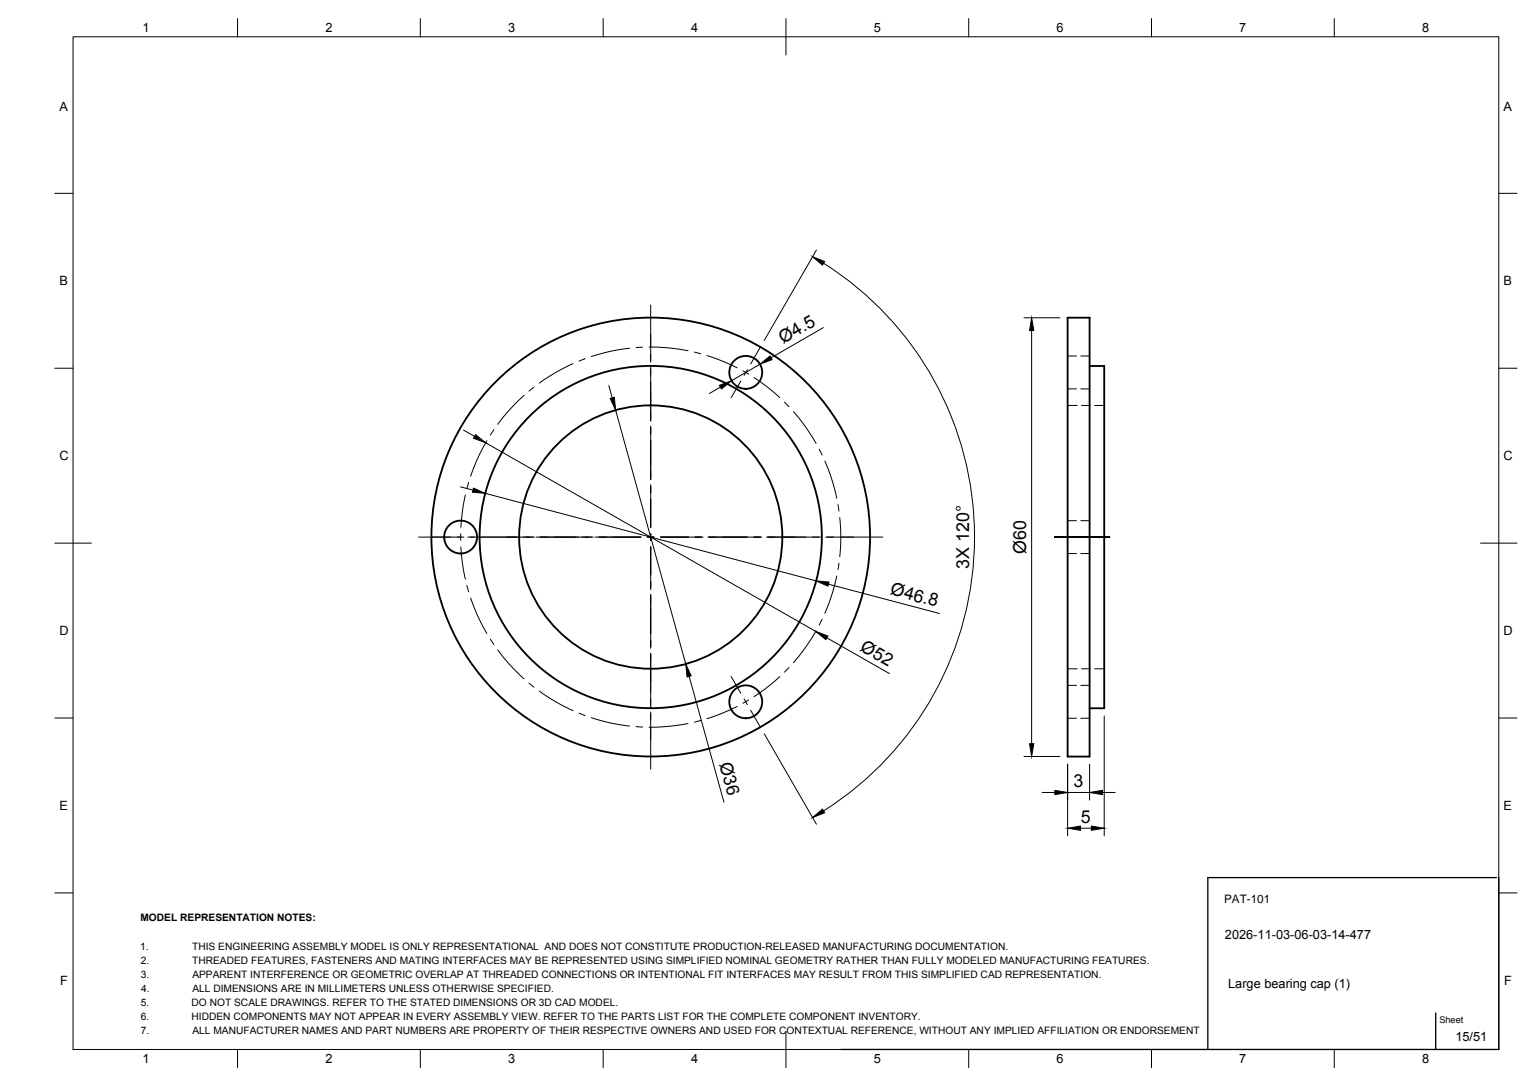
ISO-10303-21;
HEADER;
/* Generated by software containing ST-Developer
 * from STEP Tools, Inc. (www.steptools.com) 
 */

FILE_DESCRIPTION(
/* description */ ('Spur gear reduction stage 2-1 on bearing plates'),
/* implementation_level */ '2;1');

FILE_NAME(
/* name */ 'Large bearing cap (1).step',
/* time_stamp */ '2026-10-28T03:22:07-07:00',
/* author */ (''),
/* organization */ (''),
/* preprocessor_version */ 'ST-DEVELOPER v20.2',
/* originating_system */ 'Autodesk Translation Framework v15.17.0.0',
/* authorisation */ '');

FILE_SCHEMA (('AUTOMOTIVE_DESIGN { 1 0 10303 214 3 1 1 }'));
ENDSEC;

DATA;
#10=MECHANICAL_DESIGN_GEOMETRIC_PRESENTATION_REPRESENTATION('',(#957),#53909);
#871=SHAPE_REPRESENTATION_RELATIONSHIP('SRR','None',#54098,#914);
#914=ADVANCED_BREP_SHAPE_REPRESENTATION('',(#1015),#53872);
#957=STYLED_ITEM('',(#54397),#1015);
#1015=MANIFOLD_SOLID_BREP('Body1',#11281);
#1167=FACE_BOUND('',#2384,.T.);
#1168=FACE_BOUND('',#2388,.T.);
#1169=FACE_BOUND('',#2389,.T.);
#1170=FACE_BOUND('',#2390,.T.);
#1171=FACE_BOUND('',#2391,.T.);
#1172=FACE_BOUND('',#2393,.T.);
#1173=FACE_BOUND('',#2394,.T.);
#1174=FACE_BOUND('',#2395,.T.);
#1175=FACE_BOUND('',#2396,.T.);
#1289=PLANE('',#12092);
#1290=PLANE('',#12099);
#1291=PLANE('',#12100);
#1624=FACE_OUTER_BOUND('',#2379,.T.);
#1625=FACE_OUTER_BOUND('',#2380,.T.);
#1626=FACE_OUTER_BOUND('',#2381,.T.);
#1627=FACE_OUTER_BOUND('',#2382,.T.);
#1628=FACE_OUTER_BOUND('',#2383,.T.);
#1629=FACE_OUTER_BOUND('',#2385,.T.);
#1630=FACE_OUTER_BOUND('',#2386,.T.);
#1631=FACE_OUTER_BOUND('',#2387,.T.);
#1632=FACE_OUTER_BOUND('',#2392,.T.);
#2379=EDGE_LOOP('',(#7844,#7845,#7846,#7847));
#2380=EDGE_LOOP('',(#7848,#7849,#7850,#7851));
#2381=EDGE_LOOP('',(#7852,#7853,#7854,#7855));
#2382=EDGE_LOOP('',(#7856,#7857,#7858,#7859));
#2383=EDGE_LOOP('',(#7860));
#2384=EDGE_LOOP('',(#7861));
#2385=EDGE_LOOP('',(#7862,#7863,#7864,#7865));
#2386=EDGE_LOOP('',(#7866,#7867,#7868,#7869));
#2387=EDGE_LOOP('',(#7870));
#2388=EDGE_LOOP('',(#7871));
#2389=EDGE_LOOP('',(#7872));
#2390=EDGE_LOOP('',(#7873));
#2391=EDGE_LOOP('',(#7874));
#2392=EDGE_LOOP('',(#7875));
#2393=EDGE_LOOP('',(#7876));
#2394=EDGE_LOOP('',(#7877));
#2395=EDGE_LOOP('',(#7878));
#2396=EDGE_LOOP('',(#7879));
#3083=LINE('',#16523,#3724);
#3084=LINE('',#16529,#3725);
#3085=LINE('',#16535,#3726);
#3086=LINE('',#16541,#3727);
#3087=LINE('',#16549,#3728);
#3088=LINE('',#16554,#3729);
#3724=VECTOR('',#13640,0.225);
#3725=VECTOR('',#13647,0.225);
#3726=VECTOR('',#13654,0.225);
#3727=VECTOR('',#13661,2.34);
#3728=VECTOR('',#13672,1.8);
#3729=VECTOR('',#13677,3.);
#4399=CIRCLE('',#12081,0.225);
#4400=CIRCLE('',#12082,0.225);
#4401=CIRCLE('',#12084,0.225);
#4402=CIRCLE('',#12085,0.225);
#4403=CIRCLE('',#12087,0.225);
#4404=CIRCLE('',#12088,0.225);
#4405=CIRCLE('',#12090,2.34);
#4406=CIRCLE('',#12091,2.34);
#4407=CIRCLE('',#12093,1.8);
#4408=CIRCLE('',#12095,1.8);
#4409=CIRCLE('',#12097,3.);
#4410=CIRCLE('',#12098,3.);
#4948=VERTEX_POINT('',#16520);
#4949=VERTEX_POINT('',#16522);
#4950=VERTEX_POINT('',#16526);
#4951=VERTEX_POINT('',#16528);
#4952=VERTEX_POINT('',#16532);
#4953=VERTEX_POINT('',#16534);
#4954=VERTEX_POINT('',#16538);
#4955=VERTEX_POINT('',#16540);
#4956=VERTEX_POINT('',#16544);
#4957=VERTEX_POINT('',#16547);
#4958=VERTEX_POINT('',#16551);
#4959=VERTEX_POINT('',#16553);
#6064=EDGE_CURVE('',#4948,#4948,#4399,.T.);
#6065=EDGE_CURVE('',#4948,#4949,#3083,.T.);
#6066=EDGE_CURVE('',#4949,#4949,#4400,.T.);
#6067=EDGE_CURVE('',#4950,#4950,#4401,.T.);
#6068=EDGE_CURVE('',#4950,#4951,#3084,.T.);
#6069=EDGE_CURVE('',#4951,#4951,#4402,.T.);
#6070=EDGE_CURVE('',#4952,#4952,#4403,.T.);
#6071=EDGE_CURVE('',#4952,#4953,#3085,.T.);
#6072=EDGE_CURVE('',#4953,#4953,#4404,.T.);
#6073=EDGE_CURVE('',#4954,#4954,#4405,.T.);
#6074=EDGE_CURVE('',#4954,#4955,#3086,.T.);
#6075=EDGE_CURVE('',#4955,#4955,#4406,.T.);
#6076=EDGE_CURVE('',#4956,#4956,#4407,.T.);
#6077=EDGE_CURVE('',#4957,#4957,#4408,.T.);
#6078=EDGE_CURVE('',#4957,#4956,#3087,.T.);
#6079=EDGE_CURVE('',#4958,#4958,#4409,.T.);
#6080=EDGE_CURVE('',#4958,#4959,#3088,.T.);
#6081=EDGE_CURVE('',#4959,#4959,#4410,.T.);
#7844=ORIENTED_EDGE('',*,*,#6064,.F.);
#7845=ORIENTED_EDGE('',*,*,#6065,.T.);
#7846=ORIENTED_EDGE('',*,*,#6066,.F.);
#7847=ORIENTED_EDGE('',*,*,#6065,.F.);
#7848=ORIENTED_EDGE('',*,*,#6067,.F.);
#7849=ORIENTED_EDGE('',*,*,#6068,.T.);
#7850=ORIENTED_EDGE('',*,*,#6069,.F.);
#7851=ORIENTED_EDGE('',*,*,#6068,.F.);
#7852=ORIENTED_EDGE('',*,*,#6070,.F.);
#7853=ORIENTED_EDGE('',*,*,#6071,.T.);
#7854=ORIENTED_EDGE('',*,*,#6072,.F.);
#7855=ORIENTED_EDGE('',*,*,#6071,.F.);
#7856=ORIENTED_EDGE('',*,*,#6073,.F.);
#7857=ORIENTED_EDGE('',*,*,#6074,.T.);
#7858=ORIENTED_EDGE('',*,*,#6075,.T.);
#7859=ORIENTED_EDGE('',*,*,#6074,.F.);
#7860=ORIENTED_EDGE('',*,*,#6075,.F.);
#7861=ORIENTED_EDGE('',*,*,#6076,.F.);
#7862=ORIENTED_EDGE('',*,*,#6077,.F.);
#7863=ORIENTED_EDGE('',*,*,#6078,.T.);
#7864=ORIENTED_EDGE('',*,*,#6076,.T.);
#7865=ORIENTED_EDGE('',*,*,#6078,.F.);
#7866=ORIENTED_EDGE('',*,*,#6079,.F.);
#7867=ORIENTED_EDGE('',*,*,#6080,.T.);
#7868=ORIENTED_EDGE('',*,*,#6081,.T.);
#7869=ORIENTED_EDGE('',*,*,#6080,.F.);
#7870=ORIENTED_EDGE('',*,*,#6079,.T.);
#7871=ORIENTED_EDGE('',*,*,#6066,.T.);
#7872=ORIENTED_EDGE('',*,*,#6069,.T.);
#7873=ORIENTED_EDGE('',*,*,#6072,.T.);
#7874=ORIENTED_EDGE('',*,*,#6077,.T.);
#7875=ORIENTED_EDGE('',*,*,#6081,.F.);
#7876=ORIENTED_EDGE('',*,*,#6064,.T.);
#7877=ORIENTED_EDGE('',*,*,#6067,.T.);
#7878=ORIENTED_EDGE('',*,*,#6070,.T.);
#7879=ORIENTED_EDGE('',*,*,#6073,.T.);
#10490=CYLINDRICAL_SURFACE('',#12080,0.225);
#10491=CYLINDRICAL_SURFACE('',#12083,0.225);
#10492=CYLINDRICAL_SURFACE('',#12086,0.225);
#10493=CYLINDRICAL_SURFACE('',#12089,2.34);
#10494=CYLINDRICAL_SURFACE('',#12094,1.8);
#10495=CYLINDRICAL_SURFACE('',#12096,3.);
#10744=ADVANCED_FACE('',(#1624),#10490,.F.);
#10745=ADVANCED_FACE('',(#1625),#10491,.F.);
#10746=ADVANCED_FACE('',(#1626),#10492,.F.);
#10747=ADVANCED_FACE('',(#1627),#10493,.T.);
#10748=ADVANCED_FACE('',(#1628,#1167),#1289,.F.);
#10749=ADVANCED_FACE('',(#1629),#10494,.F.);
#10750=ADVANCED_FACE('',(#1630),#10495,.T.);
#10751=ADVANCED_FACE('',(#1631,#1168,#1169,#1170,#1171),#1290,.T.);
#10752=ADVANCED_FACE('',(#1632,#1172,#1173,#1174,#1175),#1291,.F.);
#11281=CLOSED_SHELL('',(#10744,#10745,#10746,#10747,#10748,#10749,#10750,
#10751,#10752));
#12079=AXIS2_PLACEMENT_3D('',#16518,#13634,#13635);
#12080=AXIS2_PLACEMENT_3D('',#16519,#13636,#13637);
#12081=AXIS2_PLACEMENT_3D('',#16521,#13638,#13639);
#12082=AXIS2_PLACEMENT_3D('',#16524,#13641,#13642);
#12083=AXIS2_PLACEMENT_3D('',#16525,#13643,#13644);
#12084=AXIS2_PLACEMENT_3D('',#16527,#13645,#13646);
#12085=AXIS2_PLACEMENT_3D('',#16530,#13648,#13649);
#12086=AXIS2_PLACEMENT_3D('',#16531,#13650,#13651);
#12087=AXIS2_PLACEMENT_3D('',#16533,#13652,#13653);
#12088=AXIS2_PLACEMENT_3D('',#16536,#13655,#13656);
#12089=AXIS2_PLACEMENT_3D('',#16537,#13657,#13658);
#12090=AXIS2_PLACEMENT_3D('',#16539,#13659,#13660);
#12091=AXIS2_PLACEMENT_3D('',#16542,#13662,#13663);
#12092=AXIS2_PLACEMENT_3D('',#16543,#13664,#13665);
#12093=AXIS2_PLACEMENT_3D('',#16545,#13666,#13667);
#12094=AXIS2_PLACEMENT_3D('',#16546,#13668,#13669);
#12095=AXIS2_PLACEMENT_3D('',#16548,#13670,#13671);
#12096=AXIS2_PLACEMENT_3D('',#16550,#13673,#13674);
#12097=AXIS2_PLACEMENT_3D('',#16552,#13675,#13676);
#12098=AXIS2_PLACEMENT_3D('',#16555,#13678,#13679);
#12099=AXIS2_PLACEMENT_3D('',#16556,#13680,#13681);
#12100=AXIS2_PLACEMENT_3D('',#16557,#13682,#13683);
#13634=DIRECTION('axis',(0.,0.,1.));
#13635=DIRECTION('refdir',(1.,0.,0.));
#13636=DIRECTION('center_axis',(0.,1.,0.));
#13637=DIRECTION('ref_axis',(1.,0.,0.));
#13638=DIRECTION('center_axis',(0.,1.,0.));
#13639=DIRECTION('ref_axis',(1.,0.,0.));
#13640=DIRECTION('',(0.,1.,0.));
#13641=DIRECTION('center_axis',(0.,-1.,0.));
#13642=DIRECTION('ref_axis',(1.,0.,0.));
#13643=DIRECTION('center_axis',(0.,1.,0.));
#13644=DIRECTION('ref_axis',(1.,0.,0.));
#13645=DIRECTION('center_axis',(0.,1.,0.));
#13646=DIRECTION('ref_axis',(1.,0.,0.));
#13647=DIRECTION('',(0.,1.,0.));
#13648=DIRECTION('center_axis',(0.,-1.,0.));
#13649=DIRECTION('ref_axis',(1.,0.,0.));
#13650=DIRECTION('center_axis',(0.,1.,0.));
#13651=DIRECTION('ref_axis',(1.,0.,0.));
#13652=DIRECTION('center_axis',(0.,1.,0.));
#13653=DIRECTION('ref_axis',(1.,0.,0.));
#13654=DIRECTION('',(0.,1.,0.));
#13655=DIRECTION('center_axis',(0.,-1.,0.));
#13656=DIRECTION('ref_axis',(1.,0.,0.));
#13657=DIRECTION('center_axis',(0.,1.,0.));
#13658=DIRECTION('ref_axis',(1.,0.,0.));
#13659=DIRECTION('center_axis',(0.,1.,0.));
#13660=DIRECTION('ref_axis',(1.,0.,0.));
#13661=DIRECTION('',(0.,-1.,0.));
#13662=DIRECTION('center_axis',(0.,1.,0.));
#13663=DIRECTION('ref_axis',(1.,0.,0.));
#13664=DIRECTION('center_axis',(0.,1.,0.));
#13665=DIRECTION('ref_axis',(1.,0.,0.));
#13666=DIRECTION('center_axis',(0.,-1.,0.));
#13667=DIRECTION('ref_axis',(1.,0.,0.));
#13668=DIRECTION('center_axis',(0.,1.,0.));
#13669=DIRECTION('ref_axis',(1.,0.,0.));
#13670=DIRECTION('center_axis',(0.,-1.,0.));
#13671=DIRECTION('ref_axis',(1.,0.,0.));
#13672=DIRECTION('',(0.,-1.,0.));
#13673=DIRECTION('center_axis',(0.,1.,0.));
#13674=DIRECTION('ref_axis',(1.,0.,0.));
#13675=DIRECTION('center_axis',(0.,1.,0.));
#13676=DIRECTION('ref_axis',(1.,0.,0.));
#13677=DIRECTION('',(0.,-1.,0.));
#13678=DIRECTION('center_axis',(0.,1.,0.));
#13679=DIRECTION('ref_axis',(1.,0.,0.));
#13680=DIRECTION('center_axis',(0.,1.,0.));
#13681=DIRECTION('ref_axis',(1.,0.,0.));
#13682=DIRECTION('center_axis',(0.,1.,0.));
#13683=DIRECTION('ref_axis',(1.,0.,0.));
#16518=CARTESIAN_POINT('',(0.,0.,0.));
#16519=CARTESIAN_POINT('Origin',(6.,4.3,7.6));
#16520=CARTESIAN_POINT('',(5.775,4.4,7.6));
#16521=CARTESIAN_POINT('Origin',(6.,4.4,7.6));
#16522=CARTESIAN_POINT('',(5.775,4.7,7.6));
#16523=CARTESIAN_POINT('',(5.775,4.3,7.6));
#16524=CARTESIAN_POINT('Origin',(6.,4.7,7.6));
#16525=CARTESIAN_POINT('Origin',(3.74833395016046,4.3,3.7));
#16526=CARTESIAN_POINT('',(3.52333395016046,4.4,3.7));
#16527=CARTESIAN_POINT('Origin',(3.74833395016046,4.4,3.7));
#16528=CARTESIAN_POINT('',(3.52333395016046,4.7,3.7));
#16529=CARTESIAN_POINT('',(3.52333395016046,4.3,3.7));
#16530=CARTESIAN_POINT('Origin',(3.74833395016046,4.7,3.7));
#16531=CARTESIAN_POINT('Origin',(8.25166604983954,4.3,3.7));
#16532=CARTESIAN_POINT('',(8.02666604983954,4.4,3.7));
#16533=CARTESIAN_POINT('Origin',(8.25166604983954,4.4,3.7));
#16534=CARTESIAN_POINT('',(8.02666604983954,4.7,3.7));
#16535=CARTESIAN_POINT('',(8.02666604983954,4.3,3.7));
#16536=CARTESIAN_POINT('Origin',(8.25166604983954,4.7,3.7));
#16537=CARTESIAN_POINT('Origin',(6.,4.2,5.));
#16538=CARTESIAN_POINT('',(3.66,4.4,5.));
#16539=CARTESIAN_POINT('Origin',(6.,4.4,5.));
#16540=CARTESIAN_POINT('',(3.66,4.2,5.));
#16541=CARTESIAN_POINT('',(3.66,4.2,5.));
#16542=CARTESIAN_POINT('Origin',(6.,4.2,5.));
#16543=CARTESIAN_POINT('Origin',(6.,4.2,5.));
#16544=CARTESIAN_POINT('',(4.2,4.2,5.));
#16545=CARTESIAN_POINT('Origin',(6.,4.2,5.));
#16546=CARTESIAN_POINT('Origin',(6.,4.4,5.));
#16547=CARTESIAN_POINT('',(4.2,4.7,5.));
#16548=CARTESIAN_POINT('Origin',(6.,4.7,5.));
#16549=CARTESIAN_POINT('',(4.2,4.4,5.));
#16550=CARTESIAN_POINT('Origin',(6.,4.4,5.));
#16551=CARTESIAN_POINT('',(3.,4.7,5.));
#16552=CARTESIAN_POINT('Origin',(6.,4.7,5.));
#16553=CARTESIAN_POINT('',(3.,4.4,5.));
#16554=CARTESIAN_POINT('',(3.,4.4,5.));
#16555=CARTESIAN_POINT('Origin',(6.,4.4,5.));
#16556=CARTESIAN_POINT('Origin',(6.,4.7,5.));
#16557=CARTESIAN_POINT('Origin',(6.,4.4,5.));
#53822=UNCERTAINTY_MEASURE_WITH_UNIT(LENGTH_MEASURE(0.001),#53910,
'DISTANCE_ACCURACY_VALUE',
'Maximum model space distance between geometric entities at asserted c
onnectivities');
#53859=UNCERTAINTY_MEASURE_WITH_UNIT(LENGTH_MEASURE(0.001),#53910,
'DISTANCE_ACCURACY_VALUE',
'Maximum model space distance between geometric entities at asserted c
onnectivities');
#53872=(
GEOMETRIC_REPRESENTATION_CONTEXT(3)
GLOBAL_UNCERTAINTY_ASSIGNED_CONTEXT((#53822))
GLOBAL_UNIT_ASSIGNED_CONTEXT((#53910,#53912,#53913))
REPRESENTATION_CONTEXT('','3D')
);
#53909=(
GEOMETRIC_REPRESENTATION_CONTEXT(3)
GLOBAL_UNCERTAINTY_ASSIGNED_CONTEXT((#53859))
GLOBAL_UNIT_ASSIGNED_CONTEXT((#53910,#53912,#53913))
REPRESENTATION_CONTEXT('','3D')
);
#53910=(
LENGTH_UNIT()
NAMED_UNIT(*)
SI_UNIT(.CENTI.,.METRE.)
);
#53912=(
NAMED_UNIT(*)
PLANE_ANGLE_UNIT()
SI_UNIT($,.RADIAN.)
);
#53913=(
NAMED_UNIT(*)
SI_UNIT($,.STERADIAN.)
SOLID_ANGLE_UNIT()
);
#53926=SHAPE_DEFINITION_REPRESENTATION(#53975,#54098);
#53975=PRODUCT_DEFINITION_SHAPE('',$,#54148);
#54098=SHAPE_REPRESENTATION('',(#12079),#53872);
#54135=PRODUCT_DEFINITION_CONTEXT('part definition',#54284,'design');
#54148=PRODUCT_DEFINITION('Large bearing cap (1)','Large bearing cap (1)',
#54197,#54135);
#54197=PRODUCT_DEFINITION_FORMATION('',$,#54298);
#54284=APPLICATION_CONTEXT(
'Core Data for Automotive Mechanical Design Process');
#54285=PRODUCT_CONTEXT('part definition',#54284,'mechanical');
#54298=PRODUCT('Large bearing cap (1)','Large bearing cap (1)',
'Large bearing cap (1)',(#54285));
#54391=COLOUR_RGB('Grey',0.48,0.52,0.57);
#54392=FILL_AREA_STYLE_COLOUR('',#54391);
#54393=FILL_AREA_STYLE('',(#54392));
#54394=SURFACE_STYLE_FILL_AREA(#54393);
#54395=SURFACE_SIDE_STYLE('',(#54394));
#54396=SURFACE_STYLE_USAGE(.BOTH.,#54395);
#54397=PRESENTATION_STYLE_ASSIGNMENT((#54396));
ENDSEC;
END-ISO-10303-21;
